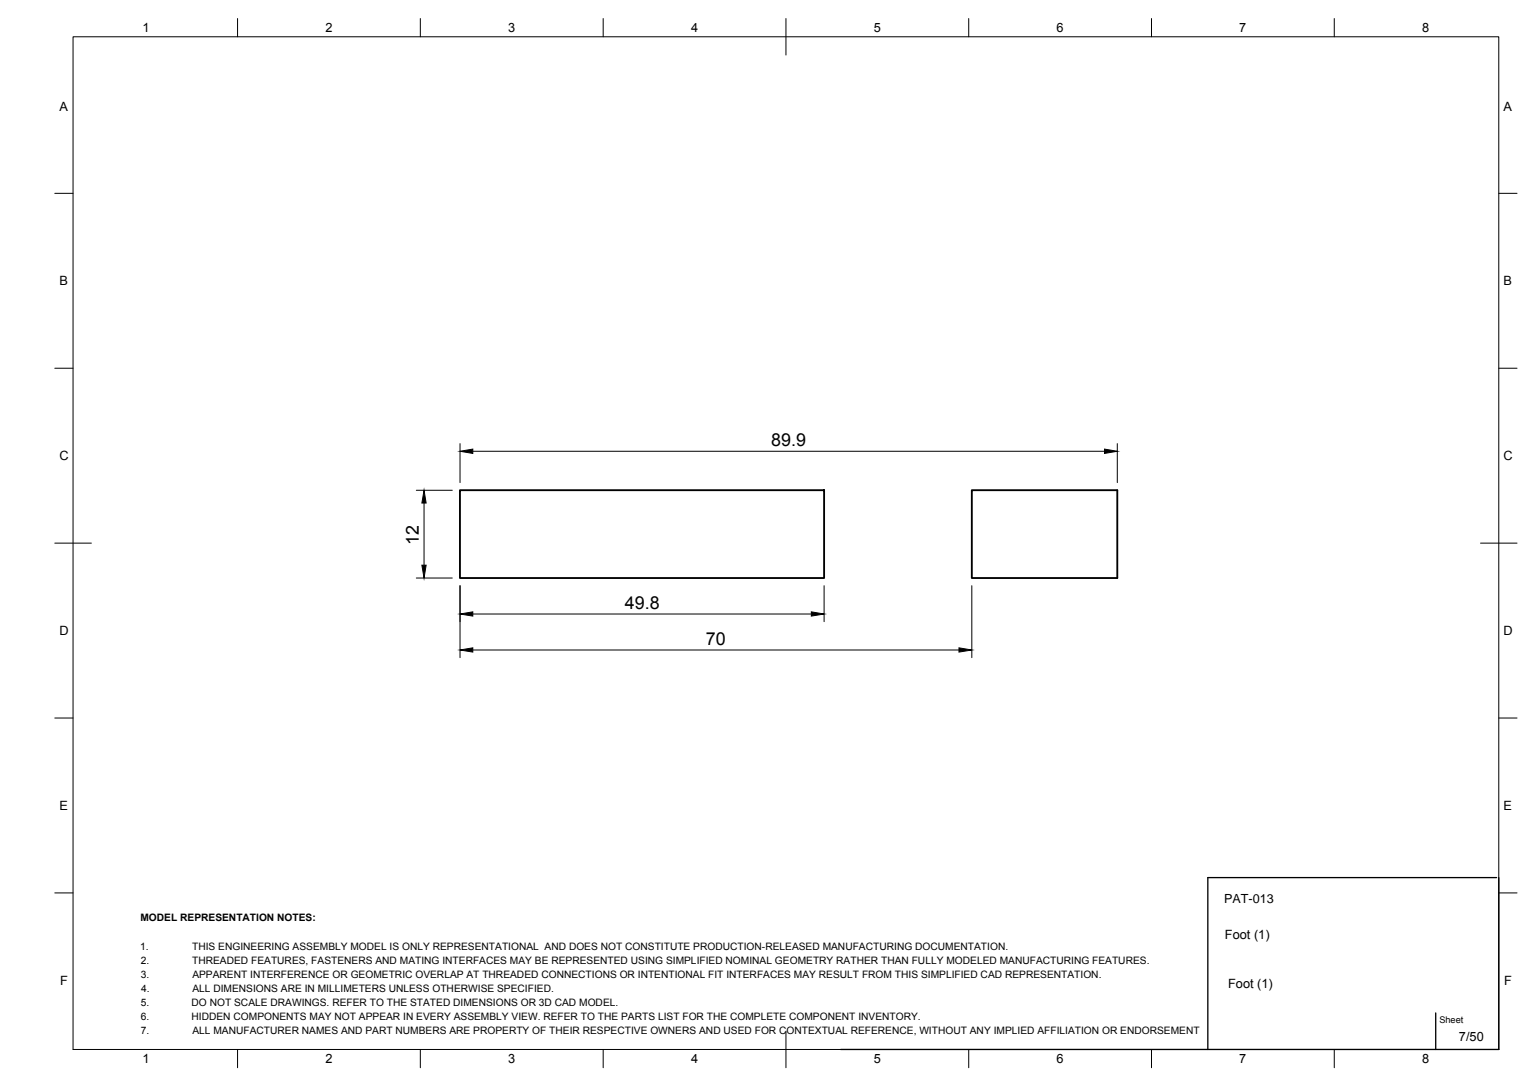
ISO-10303-21;
HEADER;
/* Generated by software containing ST-Developer
 * from STEP Tools, Inc. (www.steptools.com) 
 */

FILE_DESCRIPTION(
/* description */ ('Belt-driven linear axis on 2020 extrusion'),
/* implementation_level */ '2;1');

FILE_NAME(
/* name */ 'Foot (1).step',
/* time_stamp */ '2026-10-28T03:26:09-07:00',
/* author */ (''),
/* organization */ (''),
/* preprocessor_version */ 'ST-DEVELOPER v20.2',
/* originating_system */ 'Autodesk Translation Framework v15.17.0.0',
/* authorisation */ '');

FILE_SCHEMA (('AUTOMOTIVE_DESIGN { 1 0 10303 214 3 1 1 }'));
ENDSEC;

DATA;
#10=MECHANICAL_DESIGN_GEOMETRIC_PRESENTATION_REPRESENTATION('',(#613,#614),#20096);
#520=SHAPE_REPRESENTATION_RELATIONSHIP('SRR','None',#20316,#566);
#566=ADVANCED_BREP_SHAPE_REPRESENTATION('',(#669,#670),#20047);
#613=STYLED_ITEM('',(#20664),#669);
#614=STYLED_ITEM('',(#20664),#670);
#669=MANIFOLD_SOLID_BREP('Body1',#10926);
#670=MANIFOLD_SOLID_BREP('Body2',#10927);
#923=PLANE('',#11589);
#924=PLANE('',#11590);
#925=PLANE('',#11591);
#926=PLANE('',#11592);
#927=PLANE('',#11593);
#928=PLANE('',#11594);
#929=PLANE('',#11595);
#930=PLANE('',#11596);
#931=PLANE('',#11597);
#932=PLANE('',#11598);
#933=PLANE('',#11599);
#934=PLANE('',#11600);
#1304=FACE_OUTER_BOUND('',#1950,.T.);
#1305=FACE_OUTER_BOUND('',#1951,.T.);
#1306=FACE_OUTER_BOUND('',#1952,.T.);
#1307=FACE_OUTER_BOUND('',#1953,.T.);
#1308=FACE_OUTER_BOUND('',#1954,.T.);
#1309=FACE_OUTER_BOUND('',#1955,.T.);
#1310=FACE_OUTER_BOUND('',#1956,.T.);
#1311=FACE_OUTER_BOUND('',#1957,.T.);
#1312=FACE_OUTER_BOUND('',#1958,.T.);
#1313=FACE_OUTER_BOUND('',#1959,.T.);
#1314=FACE_OUTER_BOUND('',#1960,.T.);
#1315=FACE_OUTER_BOUND('',#1961,.T.);
#1950=EDGE_LOOP('',(#7445,#7446,#7447,#7448));
#1951=EDGE_LOOP('',(#7449,#7450,#7451,#7452));
#1952=EDGE_LOOP('',(#7453,#7454,#7455,#7456));
#1953=EDGE_LOOP('',(#7457,#7458,#7459,#7460));
#1954=EDGE_LOOP('',(#7461,#7462,#7463,#7464));
#1955=EDGE_LOOP('',(#7465,#7466,#7467,#7468));
#1956=EDGE_LOOP('',(#7469,#7470,#7471,#7472));
#1957=EDGE_LOOP('',(#7473,#7474,#7475,#7476));
#1958=EDGE_LOOP('',(#7477,#7478,#7479,#7480));
#1959=EDGE_LOOP('',(#7481,#7482,#7483,#7484));
#1960=EDGE_LOOP('',(#7485,#7486,#7487,#7488));
#1961=EDGE_LOOP('',(#7489,#7490,#7491,#7492));
#2721=LINE('',#16454,#3578);
#2722=LINE('',#16456,#3579);
#2723=LINE('',#16458,#3580);
#2724=LINE('',#16459,#3581);
#2725=LINE('',#16462,#3582);
#2726=LINE('',#16464,#3583);
#2727=LINE('',#16465,#3584);
#2728=LINE('',#16468,#3585);
#2729=LINE('',#16469,#3586);
#2730=LINE('',#16472,#3587);
#2731=LINE('',#16473,#3588);
#2732=LINE('',#16475,#3589);
#2733=LINE('',#16480,#3590);
#2734=LINE('',#16482,#3591);
#2735=LINE('',#16484,#3592);
#2736=LINE('',#16485,#3593);
#2737=LINE('',#16489,#3594);
#2738=LINE('',#16490,#3595);
#2739=LINE('',#16491,#3596);
#2740=LINE('',#16494,#3597);
#2741=LINE('',#16495,#3598);
#2742=LINE('',#16498,#3599);
#2743=LINE('',#16499,#3600);
#2744=LINE('',#16501,#3601);
#3578=VECTOR('',#13041,1.);
#3579=VECTOR('',#13042,1.);
#3580=VECTOR('',#13043,1.);
#3581=VECTOR('',#13044,1.);
#3582=VECTOR('',#13047,1.);
#3583=VECTOR('',#13048,1.);
#3584=VECTOR('',#13049,1.);
#3585=VECTOR('',#13052,1.);
#3586=VECTOR('',#13053,1.);
#3587=VECTOR('',#13056,1.);
#3588=VECTOR('',#13057,1.);
#3589=VECTOR('',#13060,1.);
#3590=VECTOR('',#13065,1.);
#3591=VECTOR('',#13066,1.);
#3592=VECTOR('',#13067,1.);
#3593=VECTOR('',#13068,1.);
#3594=VECTOR('',#13071,1.);
#3595=VECTOR('',#13072,1.);
#3596=VECTOR('',#13073,1.);
#3597=VECTOR('',#13076,1.);
#3598=VECTOR('',#13077,1.);
#3599=VECTOR('',#13080,1.);
#3600=VECTOR('',#13081,1.);
#3601=VECTOR('',#13084,1.);
#4956=VERTEX_POINT('',#16452);
#4957=VERTEX_POINT('',#16453);
#4958=VERTEX_POINT('',#16455);
#4959=VERTEX_POINT('',#16457);
#4960=VERTEX_POINT('',#16461);
#4961=VERTEX_POINT('',#16463);
#4962=VERTEX_POINT('',#16467);
#4963=VERTEX_POINT('',#16471);
#4964=VERTEX_POINT('',#16478);
#4965=VERTEX_POINT('',#16479);
#4966=VERTEX_POINT('',#16481);
#4967=VERTEX_POINT('',#16483);
#4968=VERTEX_POINT('',#16487);
#4969=VERTEX_POINT('',#16488);
#4970=VERTEX_POINT('',#16493);
#4971=VERTEX_POINT('',#16497);
#5937=EDGE_CURVE('',#4956,#4957,#2721,.T.);
#5938=EDGE_CURVE('',#4958,#4956,#2722,.T.);
#5939=EDGE_CURVE('',#4959,#4958,#2723,.T.);
#5940=EDGE_CURVE('',#4957,#4959,#2724,.T.);
#5941=EDGE_CURVE('',#4958,#4960,#2725,.T.);
#5942=EDGE_CURVE('',#4960,#4961,#2726,.T.);
#5943=EDGE_CURVE('',#4961,#4959,#2727,.T.);
#5944=EDGE_CURVE('',#4956,#4962,#2728,.T.);
#5945=EDGE_CURVE('',#4962,#4960,#2729,.T.);
#5946=EDGE_CURVE('',#4963,#4962,#2730,.T.);
#5947=EDGE_CURVE('',#4961,#4963,#2731,.T.);
#5948=EDGE_CURVE('',#4963,#4957,#2732,.T.);
#5949=EDGE_CURVE('',#4964,#4965,#2733,.T.);
#5950=EDGE_CURVE('',#4965,#4966,#2734,.T.);
#5951=EDGE_CURVE('',#4967,#4966,#2735,.T.);
#5952=EDGE_CURVE('',#4964,#4967,#2736,.T.);
#5953=EDGE_CURVE('',#4968,#4969,#2737,.T.);
#5954=EDGE_CURVE('',#4969,#4964,#2738,.T.);
#5955=EDGE_CURVE('',#4968,#4967,#2739,.T.);
#5956=EDGE_CURVE('',#4970,#4968,#2740,.T.);
#5957=EDGE_CURVE('',#4966,#4970,#2741,.T.);
#5958=EDGE_CURVE('',#4971,#4970,#2742,.T.);
#5959=EDGE_CURVE('',#4965,#4971,#2743,.T.);
#5960=EDGE_CURVE('',#4969,#4971,#2744,.T.);
#7445=ORIENTED_EDGE('',*,*,#5937,.F.);
#7446=ORIENTED_EDGE('',*,*,#5938,.F.);
#7447=ORIENTED_EDGE('',*,*,#5939,.F.);
#7448=ORIENTED_EDGE('',*,*,#5940,.F.);
#7449=ORIENTED_EDGE('',*,*,#5939,.T.);
#7450=ORIENTED_EDGE('',*,*,#5941,.T.);
#7451=ORIENTED_EDGE('',*,*,#5942,.T.);
#7452=ORIENTED_EDGE('',*,*,#5943,.T.);
#7453=ORIENTED_EDGE('',*,*,#5938,.T.);
#7454=ORIENTED_EDGE('',*,*,#5944,.T.);
#7455=ORIENTED_EDGE('',*,*,#5945,.T.);
#7456=ORIENTED_EDGE('',*,*,#5941,.F.);
#7457=ORIENTED_EDGE('',*,*,#5945,.F.);
#7458=ORIENTED_EDGE('',*,*,#5946,.F.);
#7459=ORIENTED_EDGE('',*,*,#5947,.F.);
#7460=ORIENTED_EDGE('',*,*,#5942,.F.);
#7461=ORIENTED_EDGE('',*,*,#5937,.T.);
#7462=ORIENTED_EDGE('',*,*,#5948,.F.);
#7463=ORIENTED_EDGE('',*,*,#5946,.T.);
#7464=ORIENTED_EDGE('',*,*,#5944,.F.);
#7465=ORIENTED_EDGE('',*,*,#5940,.T.);
#7466=ORIENTED_EDGE('',*,*,#5943,.F.);
#7467=ORIENTED_EDGE('',*,*,#5947,.T.);
#7468=ORIENTED_EDGE('',*,*,#5948,.T.);
#7469=ORIENTED_EDGE('',*,*,#5949,.T.);
#7470=ORIENTED_EDGE('',*,*,#5950,.T.);
#7471=ORIENTED_EDGE('',*,*,#5951,.F.);
#7472=ORIENTED_EDGE('',*,*,#5952,.F.);
#7473=ORIENTED_EDGE('',*,*,#5953,.T.);
#7474=ORIENTED_EDGE('',*,*,#5954,.T.);
#7475=ORIENTED_EDGE('',*,*,#5952,.T.);
#7476=ORIENTED_EDGE('',*,*,#5955,.F.);
#7477=ORIENTED_EDGE('',*,*,#5956,.T.);
#7478=ORIENTED_EDGE('',*,*,#5955,.T.);
#7479=ORIENTED_EDGE('',*,*,#5951,.T.);
#7480=ORIENTED_EDGE('',*,*,#5957,.T.);
#7481=ORIENTED_EDGE('',*,*,#5958,.T.);
#7482=ORIENTED_EDGE('',*,*,#5957,.F.);
#7483=ORIENTED_EDGE('',*,*,#5950,.F.);
#7484=ORIENTED_EDGE('',*,*,#5959,.T.);
#7485=ORIENTED_EDGE('',*,*,#5960,.T.);
#7486=ORIENTED_EDGE('',*,*,#5959,.F.);
#7487=ORIENTED_EDGE('',*,*,#5949,.F.);
#7488=ORIENTED_EDGE('',*,*,#5954,.F.);
#7489=ORIENTED_EDGE('',*,*,#5953,.F.);
#7490=ORIENTED_EDGE('',*,*,#5956,.F.);
#7491=ORIENTED_EDGE('',*,*,#5958,.F.);
#7492=ORIENTED_EDGE('',*,*,#5960,.F.);
#10355=ADVANCED_FACE('',(#1304),#923,.F.);
#10356=ADVANCED_FACE('',(#1305),#924,.T.);
#10357=ADVANCED_FACE('',(#1306),#925,.T.);
#10358=ADVANCED_FACE('',(#1307),#926,.F.);
#10359=ADVANCED_FACE('',(#1308),#927,.F.);
#10360=ADVANCED_FACE('',(#1309),#928,.T.);
#10361=ADVANCED_FACE('',(#1310),#929,.T.);
#10362=ADVANCED_FACE('',(#1311),#930,.T.);
#10363=ADVANCED_FACE('',(#1312),#931,.T.);
#10364=ADVANCED_FACE('',(#1313),#932,.T.);
#10365=ADVANCED_FACE('',(#1314),#933,.F.);
#10366=ADVANCED_FACE('',(#1315),#934,.F.);
#10926=CLOSED_SHELL('',(#10355,#10356,#10357,#10358,#10359,#10360));
#10927=CLOSED_SHELL('',(#10361,#10362,#10363,#10364,#10365,#10366));
#11588=AXIS2_PLACEMENT_3D('',#16450,#13037,#13038);
#11589=AXIS2_PLACEMENT_3D('',#16451,#13039,#13040);
#11590=AXIS2_PLACEMENT_3D('',#16460,#13045,#13046);
#11591=AXIS2_PLACEMENT_3D('',#16466,#13050,#13051);
#11592=AXIS2_PLACEMENT_3D('',#16470,#13054,#13055);
#11593=AXIS2_PLACEMENT_3D('',#16474,#13058,#13059);
#11594=AXIS2_PLACEMENT_3D('',#16476,#13061,#13062);
#11595=AXIS2_PLACEMENT_3D('',#16477,#13063,#13064);
#11596=AXIS2_PLACEMENT_3D('',#16486,#13069,#13070);
#11597=AXIS2_PLACEMENT_3D('',#16492,#13074,#13075);
#11598=AXIS2_PLACEMENT_3D('',#16496,#13078,#13079);
#11599=AXIS2_PLACEMENT_3D('',#16500,#13082,#13083);
#11600=AXIS2_PLACEMENT_3D('',#16502,#13085,#13086);
#13037=DIRECTION('axis',(0.,0.,1.));
#13038=DIRECTION('refdir',(1.,0.,0.));
#13039=DIRECTION('center_axis',(0.,-1.,0.));
#13040=DIRECTION('ref_axis',(1.,0.,0.));
#13041=DIRECTION('',(1.,0.,0.));
#13042=DIRECTION('',(0.,0.,-1.));
#13043=DIRECTION('',(-1.,0.,0.));
#13044=DIRECTION('',(0.,0.,1.));
#13045=DIRECTION('center_axis',(0.,0.,1.));
#13046=DIRECTION('ref_axis',(1.,0.,0.));
#13047=DIRECTION('',(0.,-1.,0.));
#13048=DIRECTION('',(1.,0.,0.));
#13049=DIRECTION('',(0.,1.,0.));
#13050=DIRECTION('center_axis',(-1.,0.,0.));
#13051=DIRECTION('ref_axis',(0.,-1.,0.));
#13052=DIRECTION('',(0.,-1.,0.));
#13053=DIRECTION('',(0.,0.,1.));
#13054=DIRECTION('center_axis',(0.,1.,0.));
#13055=DIRECTION('ref_axis',(-1.,0.,0.));
#13056=DIRECTION('',(-1.,0.,0.));
#13057=DIRECTION('',(0.,0.,-1.));
#13058=DIRECTION('center_axis',(0.,0.,1.));
#13059=DIRECTION('ref_axis',(1.,0.,0.));
#13060=DIRECTION('',(0.,1.,0.));
#13061=DIRECTION('center_axis',(1.,0.,0.));
#13062=DIRECTION('ref_axis',(0.,1.,0.));
#13063=DIRECTION('center_axis',(0.,-1.,0.));
#13064=DIRECTION('ref_axis',(1.,0.,0.));
#13065=DIRECTION('',(1.,0.,0.));
#13066=DIRECTION('',(0.,0.,1.));
#13067=DIRECTION('',(1.,0.,0.));
#13068=DIRECTION('',(0.,0.,1.));
#13069=DIRECTION('center_axis',(-1.,0.,0.));
#13070=DIRECTION('ref_axis',(0.,-1.,0.));
#13071=DIRECTION('',(0.,0.,-1.));
#13072=DIRECTION('',(0.,-1.,0.));
#13073=DIRECTION('',(0.,-1.,0.));
#13074=DIRECTION('center_axis',(0.,0.,1.));
#13075=DIRECTION('ref_axis',(1.,0.,0.));
#13076=DIRECTION('',(-1.,0.,0.));
#13077=DIRECTION('',(0.,1.,0.));
#13078=DIRECTION('center_axis',(1.,0.,0.));
#13079=DIRECTION('ref_axis',(0.,1.,0.));
#13080=DIRECTION('',(0.,0.,1.));
#13081=DIRECTION('',(0.,1.,0.));
#13082=DIRECTION('center_axis',(0.,0.,1.));
#13083=DIRECTION('ref_axis',(1.,0.,0.));
#13084=DIRECTION('',(1.,0.,0.));
#13085=DIRECTION('center_axis',(0.,-1.,0.));
#13086=DIRECTION('ref_axis',(1.,0.,0.));
#16450=CARTESIAN_POINT('',(0.,0.,0.));
#16451=CARTESIAN_POINT('Origin',(-4.1,2.49,-2.5));
#16452=CARTESIAN_POINT('',(35.,2.49,-2.4));
#16453=CARTESIAN_POINT('',(36.,2.49,-2.4));
#16454=CARTESIAN_POINT('',(15.7,2.49,-2.4));
#16455=CARTESIAN_POINT('',(35.,2.49,-1.2));
#16456=CARTESIAN_POINT('',(35.,2.49,-2.45));
#16457=CARTESIAN_POINT('',(36.,2.49,-1.2));
#16458=CARTESIAN_POINT('',(15.7,2.49,-1.2));
#16459=CARTESIAN_POINT('',(36.,2.49,-2.45));
#16460=CARTESIAN_POINT('Origin',(35.5,-1.,-1.2));
#16461=CARTESIAN_POINT('',(35.,-2.49,-1.2));
#16462=CARTESIAN_POINT('',(35.,4.5,-1.2));
#16463=CARTESIAN_POINT('',(36.,-2.49,-1.2));
#16464=CARTESIAN_POINT('',(35.8,-2.49,-1.2));
#16465=CARTESIAN_POINT('',(36.,-6.5,-1.2));
#16466=CARTESIAN_POINT('Origin',(35.,4.5,-2.4));
#16467=CARTESIAN_POINT('',(35.,-2.49,-2.4));
#16468=CARTESIAN_POINT('',(35.,4.5,-2.4));
#16469=CARTESIAN_POINT('',(35.,-2.49,-2.45));
#16470=CARTESIAN_POINT('Origin',(36.1,-2.49,-2.5));
#16471=CARTESIAN_POINT('',(36.,-2.49,-2.4));
#16472=CARTESIAN_POINT('',(35.8,-2.49,-2.4));
#16473=CARTESIAN_POINT('',(36.,-2.49,-2.45));
#16474=CARTESIAN_POINT('Origin',(35.5,-1.,-2.4));
#16475=CARTESIAN_POINT('',(36.,-6.5,-2.4));
#16476=CARTESIAN_POINT('Origin',(36.,-6.5,-2.4));
#16477=CARTESIAN_POINT('Origin',(35.,-6.5,-2.4));
#16478=CARTESIAN_POINT('',(35.,-6.5,-2.4));
#16479=CARTESIAN_POINT('',(36.,-6.5,-2.4));
#16480=CARTESIAN_POINT('',(35.,-6.5,-2.4));
#16481=CARTESIAN_POINT('',(36.,-6.5,-1.2));
#16482=CARTESIAN_POINT('',(36.,-6.5,-2.4));
#16483=CARTESIAN_POINT('',(35.,-6.5,-1.2));
#16484=CARTESIAN_POINT('',(35.,-6.5,-1.2));
#16485=CARTESIAN_POINT('',(35.,-6.5,-2.4));
#16486=CARTESIAN_POINT('Origin',(35.,4.5,-2.4));
#16487=CARTESIAN_POINT('',(35.,-4.51,-1.2));
#16488=CARTESIAN_POINT('',(35.,-4.51,-2.4));
#16489=CARTESIAN_POINT('',(35.,-4.51,-2.45));
#16490=CARTESIAN_POINT('',(35.,4.5,-2.4));
#16491=CARTESIAN_POINT('',(35.,4.5,-1.2));
#16492=CARTESIAN_POINT('Origin',(35.5,-1.,-1.2));
#16493=CARTESIAN_POINT('',(36.,-4.51,-1.2));
#16494=CARTESIAN_POINT('',(15.7,-4.51,-1.2));
#16495=CARTESIAN_POINT('',(36.,-6.5,-1.2));
#16496=CARTESIAN_POINT('Origin',(36.,-6.5,-2.4));
#16497=CARTESIAN_POINT('',(36.,-4.51,-2.4));
#16498=CARTESIAN_POINT('',(36.,-4.51,-2.45));
#16499=CARTESIAN_POINT('',(36.,-6.5,-2.4));
#16500=CARTESIAN_POINT('Origin',(35.5,-1.,-2.4));
#16501=CARTESIAN_POINT('',(15.7,-4.51,-2.4));
#16502=CARTESIAN_POINT('Origin',(-4.1,-4.51,-2.5));
#19993=UNCERTAINTY_MEASURE_WITH_UNIT(LENGTH_MEASURE(0.001),#20097,
'DISTANCE_ACCURACY_VALUE',
'Maximum model space distance between geometric entities at asserted c
onnectivities');
#20042=UNCERTAINTY_MEASURE_WITH_UNIT(LENGTH_MEASURE(0.001),#20097,
'DISTANCE_ACCURACY_VALUE',
'Maximum model space distance between geometric entities at asserted c
onnectivities');
#20047=(
GEOMETRIC_REPRESENTATION_CONTEXT(3)
GLOBAL_UNCERTAINTY_ASSIGNED_CONTEXT((#19993))
GLOBAL_UNIT_ASSIGNED_CONTEXT((#20097,#20099,#20100))
REPRESENTATION_CONTEXT('','3D')
);
#20096=(
GEOMETRIC_REPRESENTATION_CONTEXT(3)
GLOBAL_UNCERTAINTY_ASSIGNED_CONTEXT((#20042))
GLOBAL_UNIT_ASSIGNED_CONTEXT((#20097,#20099,#20100))
REPRESENTATION_CONTEXT('','3D')
);
#20097=(
LENGTH_UNIT()
NAMED_UNIT(*)
SI_UNIT(.CENTI.,.METRE.)
);
#20099=(
NAMED_UNIT(*)
PLANE_ANGLE_UNIT()
SI_UNIT($,.RADIAN.)
);
#20100=(
NAMED_UNIT(*)
SI_UNIT($,.STERADIAN.)
SOLID_ANGLE_UNIT()
);
#20105=SHAPE_DEFINITION_REPRESENTATION(#20158,#20316);
#20158=PRODUCT_DEFINITION_SHAPE('',$,#20370);
#20316=SHAPE_REPRESENTATION('',(#11588),#20047);
#20365=PRODUCT_DEFINITION_CONTEXT('part definition',#20526,'design');
#20370=PRODUCT_DEFINITION('Foot (1)','Foot (1)',#20423,#20365);
#20423=PRODUCT_DEFINITION_FORMATION('',$,#20532);
#20526=APPLICATION_CONTEXT(
'Core Data for Automotive Mechanical Design Process');
#20527=PRODUCT_CONTEXT('part definition',#20526,'mechanical');
#20532=PRODUCT('Foot (1)','Foot (1)','Foot (1)',(#20527));
#20658=COLOUR_RGB('Off White',0.89,0.88,0.83);
#20659=FILL_AREA_STYLE_COLOUR('',#20658);
#20660=FILL_AREA_STYLE('',(#20659));
#20661=SURFACE_STYLE_FILL_AREA(#20660);
#20662=SURFACE_SIDE_STYLE('',(#20661));
#20663=SURFACE_STYLE_USAGE(.BOTH.,#20662);
#20664=PRESENTATION_STYLE_ASSIGNMENT((#20663));
ENDSEC;
END-ISO-10303-21;
